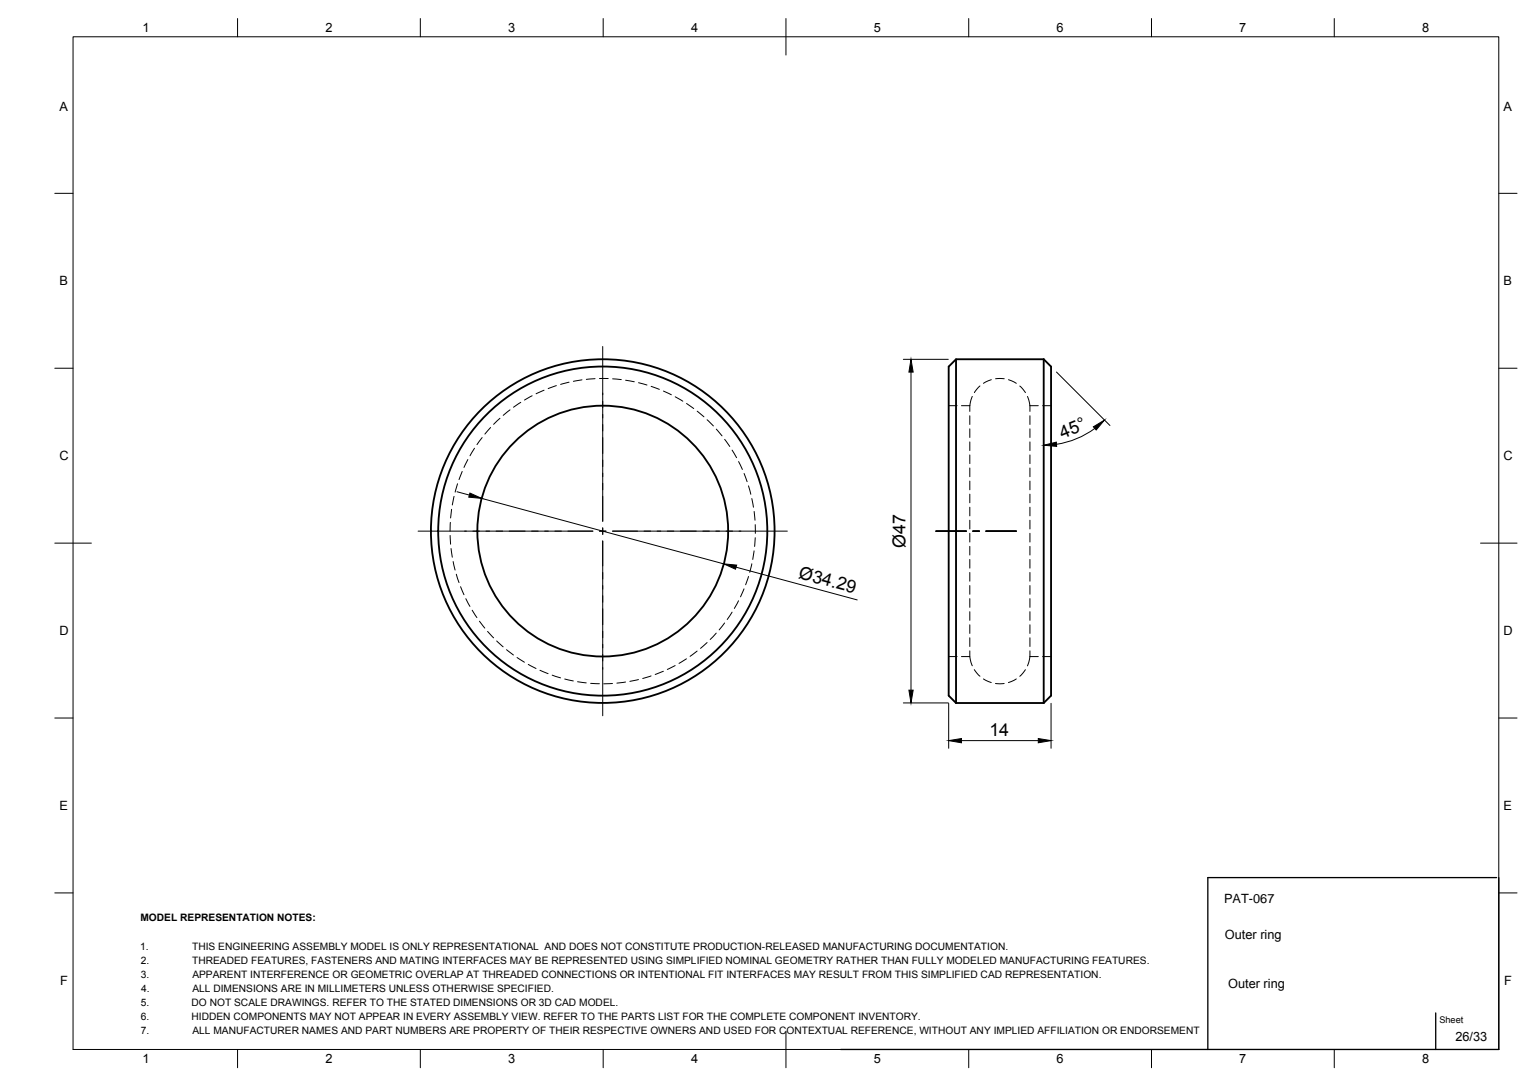
ISO-10303-21;
HEADER;
/* Generated by software containing ST-Developer
 * from STEP Tools, Inc. (www.steptools.com) 
 */

FILE_DESCRIPTION(
/* description */ ('Lifting hook block with sheave'),
/* implementation_level */ '2;1');

FILE_NAME(
/* name */ 'Outer ring.step',
/* time_stamp */ '2026-10-28T03:23:54-07:00',
/* author */ (''),
/* organization */ (''),
/* preprocessor_version */ 'ST-DEVELOPER v20.2',
/* originating_system */ 'Autodesk Translation Framework v15.17.0.0',
/* authorisation */ '');

FILE_SCHEMA (('AUTOMOTIVE_DESIGN { 1 0 10303 214 3 1 1 }'));
ENDSEC;

DATA;
#10=MECHANICAL_DESIGN_GEOMETRIC_PRESENTATION_REPRESENTATION('',(#372),#9391);
#46=TOROIDAL_SURFACE('',#5704,1.675,0.412776);
#280=CONICAL_SURFACE('',#5715,2.3,0.785398163397449);
#281=CONICAL_SURFACE('',#5719,2.3,0.785398163397449);
#312=SHAPE_REPRESENTATION_RELATIONSHIP('SRR','None',#9545,#342);
#342=ADVANCED_BREP_SHAPE_REPRESENTATION('',(#408),#9380);
#372=STYLED_ITEM('',(#9759),#408);
#408=MANIFOLD_SOLID_BREP('Body1',#4910);
#631=LINE('',#8532,#919);
#632=LINE('',#8541,#920);
#633=LINE('',#8545,#921);
#634=LINE('',#8549,#922);
#635=LINE('',#8552,#923);
#919=VECTOR('',#7042,1.71469);
#920=VECTOR('',#7053,2.3);
#921=VECTOR('',#7058,2.35);
#922=VECTOR('',#7063,2.3);
#923=VECTOR('',#7068,1.71469);
#1084=CYLINDRICAL_SURFACE('',#5710,1.71469);
#1085=CYLINDRICAL_SURFACE('',#5717,2.35);
#1086=CYLINDRICAL_SURFACE('',#5722,1.71469);
#1204=FACE_BOUND('',#1806,.T.);
#1205=FACE_BOUND('',#1811,.T.);
#1417=FACE_OUTER_BOUND('',#1803,.T.);
#1418=FACE_OUTER_BOUND('',#1804,.T.);
#1419=FACE_OUTER_BOUND('',#1805,.T.);
#1420=FACE_OUTER_BOUND('',#1807,.T.);
#1421=FACE_OUTER_BOUND('',#1808,.T.);
#1422=FACE_OUTER_BOUND('',#1809,.T.);
#1423=FACE_OUTER_BOUND('',#1810,.T.);
#1424=FACE_OUTER_BOUND('',#1812,.T.);
#1803=EDGE_LOOP('',(#4066,#4067,#4068,#4069,#4070,#4071));
#1804=EDGE_LOOP('',(#4072,#4073,#4074,#4075,#4076));
#1805=EDGE_LOOP('',(#4077));
#1806=EDGE_LOOP('',(#4078));
#1807=EDGE_LOOP('',(#4079,#4080,#4081,#4082));
#1808=EDGE_LOOP('',(#4083,#4084,#4085,#4086));
#1809=EDGE_LOOP('',(#4087,#4088,#4089,#4090));
#1810=EDGE_LOOP('',(#4091));
#1811=EDGE_LOOP('',(#4092));
#1812=EDGE_LOOP('',(#4093,#4094,#4095,#4096,#4097));
#2114=CIRCLE('',#5705,1.71469);
#2115=CIRCLE('',#5706,1.71469);
#2116=CIRCLE('',#5707,0.412776);
#2117=CIRCLE('',#5708,1.71469);
#2118=CIRCLE('',#5709,1.71469);
#2119=CIRCLE('',#5711,1.71469);
#2120=CIRCLE('',#5713,2.25);
#2121=CIRCLE('',#5714,1.71469);
#2122=CIRCLE('',#5716,2.35);
#2123=CIRCLE('',#5718,2.35);
#2124=CIRCLE('',#5720,2.25);
#2482=VERTEX_POINT('',#8520);
#2483=VERTEX_POINT('',#8521);
#2484=VERTEX_POINT('',#8524);
#2485=VERTEX_POINT('',#8526);
#2486=VERTEX_POINT('',#8530);
#2487=VERTEX_POINT('',#8534);
#2488=VERTEX_POINT('',#8536);
#2489=VERTEX_POINT('',#8539);
#2490=VERTEX_POINT('',#8543);
#2491=VERTEX_POINT('',#8547);
#3037=EDGE_CURVE('',#2482,#2483,#2114,.T.);
#3038=EDGE_CURVE('',#2483,#2482,#2115,.T.);
#3039=EDGE_CURVE('',#2483,#2484,#2116,.T.);
#3040=EDGE_CURVE('',#2485,#2484,#2117,.T.);
#3041=EDGE_CURVE('',#2484,#2485,#2118,.T.);
#3042=EDGE_CURVE('',#2486,#2486,#2119,.T.);
#3043=EDGE_CURVE('',#2486,#2485,#631,.T.);
#3044=EDGE_CURVE('',#2487,#2487,#2120,.T.);
#3045=EDGE_CURVE('',#2488,#2488,#2121,.T.);
#3046=EDGE_CURVE('',#2489,#2489,#2122,.T.);
#3047=EDGE_CURVE('',#2489,#2487,#632,.T.);
#3048=EDGE_CURVE('',#2490,#2490,#2123,.T.);
#3049=EDGE_CURVE('',#2490,#2489,#633,.T.);
#3050=EDGE_CURVE('',#2491,#2491,#2124,.T.);
#3051=EDGE_CURVE('',#2491,#2490,#634,.T.);
#3052=EDGE_CURVE('',#2482,#2488,#635,.T.);
#4066=ORIENTED_EDGE('',*,*,#3037,.F.);
#4067=ORIENTED_EDGE('',*,*,#3038,.F.);
#4068=ORIENTED_EDGE('',*,*,#3039,.T.);
#4069=ORIENTED_EDGE('',*,*,#3040,.F.);
#4070=ORIENTED_EDGE('',*,*,#3041,.F.);
#4071=ORIENTED_EDGE('',*,*,#3039,.F.);
#4072=ORIENTED_EDGE('',*,*,#3042,.T.);
#4073=ORIENTED_EDGE('',*,*,#3043,.T.);
#4074=ORIENTED_EDGE('',*,*,#3040,.T.);
#4075=ORIENTED_EDGE('',*,*,#3041,.T.);
#4076=ORIENTED_EDGE('',*,*,#3043,.F.);
#4077=ORIENTED_EDGE('',*,*,#3044,.F.);
#4078=ORIENTED_EDGE('',*,*,#3045,.T.);
#4079=ORIENTED_EDGE('',*,*,#3046,.F.);
#4080=ORIENTED_EDGE('',*,*,#3047,.T.);
#4081=ORIENTED_EDGE('',*,*,#3044,.T.);
#4082=ORIENTED_EDGE('',*,*,#3047,.F.);
#4083=ORIENTED_EDGE('',*,*,#3048,.F.);
#4084=ORIENTED_EDGE('',*,*,#3049,.T.);
#4085=ORIENTED_EDGE('',*,*,#3046,.T.);
#4086=ORIENTED_EDGE('',*,*,#3049,.F.);
#4087=ORIENTED_EDGE('',*,*,#3050,.F.);
#4088=ORIENTED_EDGE('',*,*,#3051,.T.);
#4089=ORIENTED_EDGE('',*,*,#3048,.T.);
#4090=ORIENTED_EDGE('',*,*,#3051,.F.);
#4091=ORIENTED_EDGE('',*,*,#3050,.T.);
#4092=ORIENTED_EDGE('',*,*,#3042,.F.);
#4093=ORIENTED_EDGE('',*,*,#3037,.T.);
#4094=ORIENTED_EDGE('',*,*,#3038,.T.);
#4095=ORIENTED_EDGE('',*,*,#3052,.T.);
#4096=ORIENTED_EDGE('',*,*,#3045,.F.);
#4097=ORIENTED_EDGE('',*,*,#3052,.F.);
#4549=PLANE('',#5712);
#4550=PLANE('',#5721);
#4793=ADVANCED_FACE('',(#1417),#46,.F.);
#4794=ADVANCED_FACE('',(#1418),#1084,.F.);
#4795=ADVANCED_FACE('',(#1419,#1204),#4549,.T.);
#4796=ADVANCED_FACE('',(#1420),#280,.T.);
#4797=ADVANCED_FACE('',(#1421),#1085,.T.);
#4798=ADVANCED_FACE('',(#1422),#281,.T.);
#4799=ADVANCED_FACE('',(#1423,#1205),#4550,.T.);
#4800=ADVANCED_FACE('',(#1424),#1086,.F.);
#4910=CLOSED_SHELL('',(#4793,#4794,#4795,#4796,#4797,#4798,#4799,#4800));
#5703=AXIS2_PLACEMENT_3D('',#8518,#7024,#7025);
#5704=AXIS2_PLACEMENT_3D('',#8519,#7026,#7027);
#5705=AXIS2_PLACEMENT_3D('',#8522,#7028,#7029);
#5706=AXIS2_PLACEMENT_3D('',#8523,#7030,#7031);
#5707=AXIS2_PLACEMENT_3D('',#8525,#7032,#7033);
#5708=AXIS2_PLACEMENT_3D('',#8527,#7034,#7035);
#5709=AXIS2_PLACEMENT_3D('',#8528,#7036,#7037);
#5710=AXIS2_PLACEMENT_3D('',#8529,#7038,#7039);
#5711=AXIS2_PLACEMENT_3D('',#8531,#7040,#7041);
#5712=AXIS2_PLACEMENT_3D('',#8533,#7043,#7044);
#5713=AXIS2_PLACEMENT_3D('',#8535,#7045,#7046);
#5714=AXIS2_PLACEMENT_3D('',#8537,#7047,#7048);
#5715=AXIS2_PLACEMENT_3D('',#8538,#7049,#7050);
#5716=AXIS2_PLACEMENT_3D('',#8540,#7051,#7052);
#5717=AXIS2_PLACEMENT_3D('',#8542,#7054,#7055);
#5718=AXIS2_PLACEMENT_3D('',#8544,#7056,#7057);
#5719=AXIS2_PLACEMENT_3D('',#8546,#7059,#7060);
#5720=AXIS2_PLACEMENT_3D('',#8548,#7061,#7062);
#5721=AXIS2_PLACEMENT_3D('',#8550,#7064,#7065);
#5722=AXIS2_PLACEMENT_3D('',#8551,#7066,#7067);
#7024=DIRECTION('axis',(0.,0.,1.));
#7025=DIRECTION('refdir',(1.,0.,0.));
#7026=DIRECTION('center_axis',(0.,-1.,0.));
#7027=DIRECTION('ref_axis',(0.,0.,-1.));
#7028=DIRECTION('center_axis',(0.,-1.,0.));
#7029=DIRECTION('ref_axis',(1.,0.,0.));
#7030=DIRECTION('center_axis',(0.,-1.,0.));
#7031=DIRECTION('ref_axis',(1.,0.,0.));
#7032=DIRECTION('center_axis',(1.,0.,1.22464679914735E-16));
#7033=DIRECTION('ref_axis',(-1.22464679914735E-16,0.,1.));
#7034=DIRECTION('center_axis',(0.,1.,0.));
#7035=DIRECTION('ref_axis',(1.,0.,0.));
#7036=DIRECTION('center_axis',(0.,1.,0.));
#7037=DIRECTION('ref_axis',(1.,0.,0.));
#7038=DIRECTION('center_axis',(0.,-1.,0.));
#7039=DIRECTION('ref_axis',(1.,0.,0.));
#7040=DIRECTION('center_axis',(0.,-1.,0.));
#7041=DIRECTION('ref_axis',(1.,0.,0.));
#7042=DIRECTION('',(0.,1.,0.));
#7043=DIRECTION('center_axis',(0.,1.,0.));
#7044=DIRECTION('ref_axis',(0.,0.,1.));
#7045=DIRECTION('center_axis',(0.,-1.,0.));
#7046=DIRECTION('ref_axis',(1.,0.,0.));
#7047=DIRECTION('center_axis',(0.,-1.,0.));
#7048=DIRECTION('ref_axis',(1.,0.,0.));
#7049=DIRECTION('center_axis',(0.,-1.,0.));
#7050=DIRECTION('ref_axis',(1.,0.,0.));
#7051=DIRECTION('center_axis',(0.,-1.,0.));
#7052=DIRECTION('ref_axis',(1.,0.,0.));
#7053=DIRECTION('',(0.707106781186548,0.707106781186547,8.65956056235494E-17));
#7054=DIRECTION('center_axis',(0.,-1.,0.));
#7055=DIRECTION('ref_axis',(1.,0.,0.));
#7056=DIRECTION('center_axis',(0.,-1.,0.));
#7057=DIRECTION('ref_axis',(1.,0.,0.));
#7058=DIRECTION('',(0.,1.,0.));
#7059=DIRECTION('center_axis',(0.,1.,0.));
#7060=DIRECTION('ref_axis',(1.,0.,0.));
#7061=DIRECTION('center_axis',(0.,-1.,0.));
#7062=DIRECTION('ref_axis',(1.,0.,0.));
#7063=DIRECTION('',(-0.707106781186548,0.707106781186547,-8.65956056235494E-17));
#7064=DIRECTION('center_axis',(0.,-1.,0.));
#7065=DIRECTION('ref_axis',(0.,0.,-1.));
#7066=DIRECTION('center_axis',(0.,-1.,0.));
#7067=DIRECTION('ref_axis',(1.,0.,0.));
#7068=DIRECTION('',(0.,1.,0.));
#8518=CARTESIAN_POINT('',(0.,0.,0.));
#8519=CARTESIAN_POINT('Origin',(0.,0.,0.));
#8520=CARTESIAN_POINT('',(-1.71469,0.410863395882378,-2.09988962002998E-16));
#8521=CARTESIAN_POINT('',(-2.09988962002998E-16,0.410863395882378,1.71469));
#8522=CARTESIAN_POINT('Origin',(0.,0.410863395882378,0.));
#8523=CARTESIAN_POINT('Origin',(0.,0.410863395882378,0.));
#8524=CARTESIAN_POINT('',(-2.09988962002998E-16,-0.410863395882378,1.71469));
#8525=CARTESIAN_POINT('Origin',(-2.05128338857182E-16,0.,1.675));
#8526=CARTESIAN_POINT('',(-1.71469,-0.410863395882378,2.09988962002998E-16));
#8527=CARTESIAN_POINT('Origin',(0.,-0.410863395882378,0.));
#8528=CARTESIAN_POINT('Origin',(0.,-0.410863395882378,0.));
#8529=CARTESIAN_POINT('Origin',(0.,0.,0.));
#8530=CARTESIAN_POINT('',(-1.71469,-0.7,-2.09988962002998E-16));
#8531=CARTESIAN_POINT('Origin',(0.,-0.7,0.));
#8532=CARTESIAN_POINT('',(-1.71469,0.,-2.09988962002998E-16));
#8533=CARTESIAN_POINT('Origin',(2.25,0.7,0.));
#8534=CARTESIAN_POINT('',(-2.25,0.7,-2.75545529808154E-16));
#8535=CARTESIAN_POINT('Origin',(0.,0.7,0.));
#8536=CARTESIAN_POINT('',(-1.71469,0.7,-2.09988962002998E-16));
#8537=CARTESIAN_POINT('Origin',(0.,0.7,0.));
#8538=CARTESIAN_POINT('Origin',(0.,0.65,0.));
#8539=CARTESIAN_POINT('',(-2.35,0.6,-2.87791997799628E-16));
#8540=CARTESIAN_POINT('Origin',(0.,0.6,0.));
#8541=CARTESIAN_POINT('',(-2.3,0.65,-2.81668763803891E-16));
#8542=CARTESIAN_POINT('Origin',(0.,0.,0.));
#8543=CARTESIAN_POINT('',(-2.35,-0.6,-2.87791997799628E-16));
#8544=CARTESIAN_POINT('Origin',(0.,-0.6,0.));
#8545=CARTESIAN_POINT('',(-2.35,0.,-2.87791997799628E-16));
#8546=CARTESIAN_POINT('Origin',(0.,-0.65,0.));
#8547=CARTESIAN_POINT('',(-2.25,-0.7,-2.75545529808154E-16));
#8548=CARTESIAN_POINT('Origin',(0.,-0.7,0.));
#8549=CARTESIAN_POINT('',(-2.3,-0.65,-2.81668763803891E-16));
#8550=CARTESIAN_POINT('Origin',(1.71469,-0.7,0.));
#8551=CARTESIAN_POINT('Origin',(0.,0.,0.));
#8552=CARTESIAN_POINT('',(-1.71469,0.,-2.09988962002998E-16));
#9343=UNCERTAINTY_MEASURE_WITH_UNIT(LENGTH_MEASURE(0.001),#9392,
'DISTANCE_ACCURACY_VALUE',
'Maximum model space distance between geometric entities at asserted c
onnectivities');
#9354=UNCERTAINTY_MEASURE_WITH_UNIT(LENGTH_MEASURE(0.001),#9392,
'DISTANCE_ACCURACY_VALUE',
'Maximum model space distance between geometric entities at asserted c
onnectivities');
#9380=(
GEOMETRIC_REPRESENTATION_CONTEXT(3)
GLOBAL_UNCERTAINTY_ASSIGNED_CONTEXT((#9343))
GLOBAL_UNIT_ASSIGNED_CONTEXT((#9392,#9394,#9395))
REPRESENTATION_CONTEXT('','3D')
);
#9391=(
GEOMETRIC_REPRESENTATION_CONTEXT(3)
GLOBAL_UNCERTAINTY_ASSIGNED_CONTEXT((#9354))
GLOBAL_UNIT_ASSIGNED_CONTEXT((#9392,#9394,#9395))
REPRESENTATION_CONTEXT('','3D')
);
#9392=(
LENGTH_UNIT()
NAMED_UNIT(*)
SI_UNIT(.CENTI.,.METRE.)
);
#9394=(
NAMED_UNIT(*)
PLANE_ANGLE_UNIT()
SI_UNIT($,.RADIAN.)
);
#9395=(
NAMED_UNIT(*)
SI_UNIT($,.STERADIAN.)
SOLID_ANGLE_UNIT()
);
#9421=SHAPE_DEFINITION_REPRESENTATION(#9482,#9545);
#9482=PRODUCT_DEFINITION_SHAPE('',$,#9582);
#9545=SHAPE_REPRESENTATION('',(#5703),#9380);
#9556=PRODUCT_DEFINITION_CONTEXT('part definition',#9666,'design');
#9582=PRODUCT_DEFINITION('Outer ring','Outer ring',#9618,#9556);
#9618=PRODUCT_DEFINITION_FORMATION('',$,#9693);
#9666=APPLICATION_CONTEXT(
'Core Data for Automotive Mechanical Design Process');
#9667=PRODUCT_CONTEXT('part definition',#9666,'mechanical');
#9693=PRODUCT('Outer ring','Outer ring','Outer ring',(#9667));
#9753=COLOUR_RGB('Grey',0.48,0.52,0.57);
#9754=FILL_AREA_STYLE_COLOUR('',#9753);
#9755=FILL_AREA_STYLE('',(#9754));
#9756=SURFACE_STYLE_FILL_AREA(#9755);
#9757=SURFACE_SIDE_STYLE('',(#9756));
#9758=SURFACE_STYLE_USAGE(.BOTH.,#9757);
#9759=PRESENTATION_STYLE_ASSIGNMENT((#9758));
ENDSEC;
END-ISO-10303-21;
